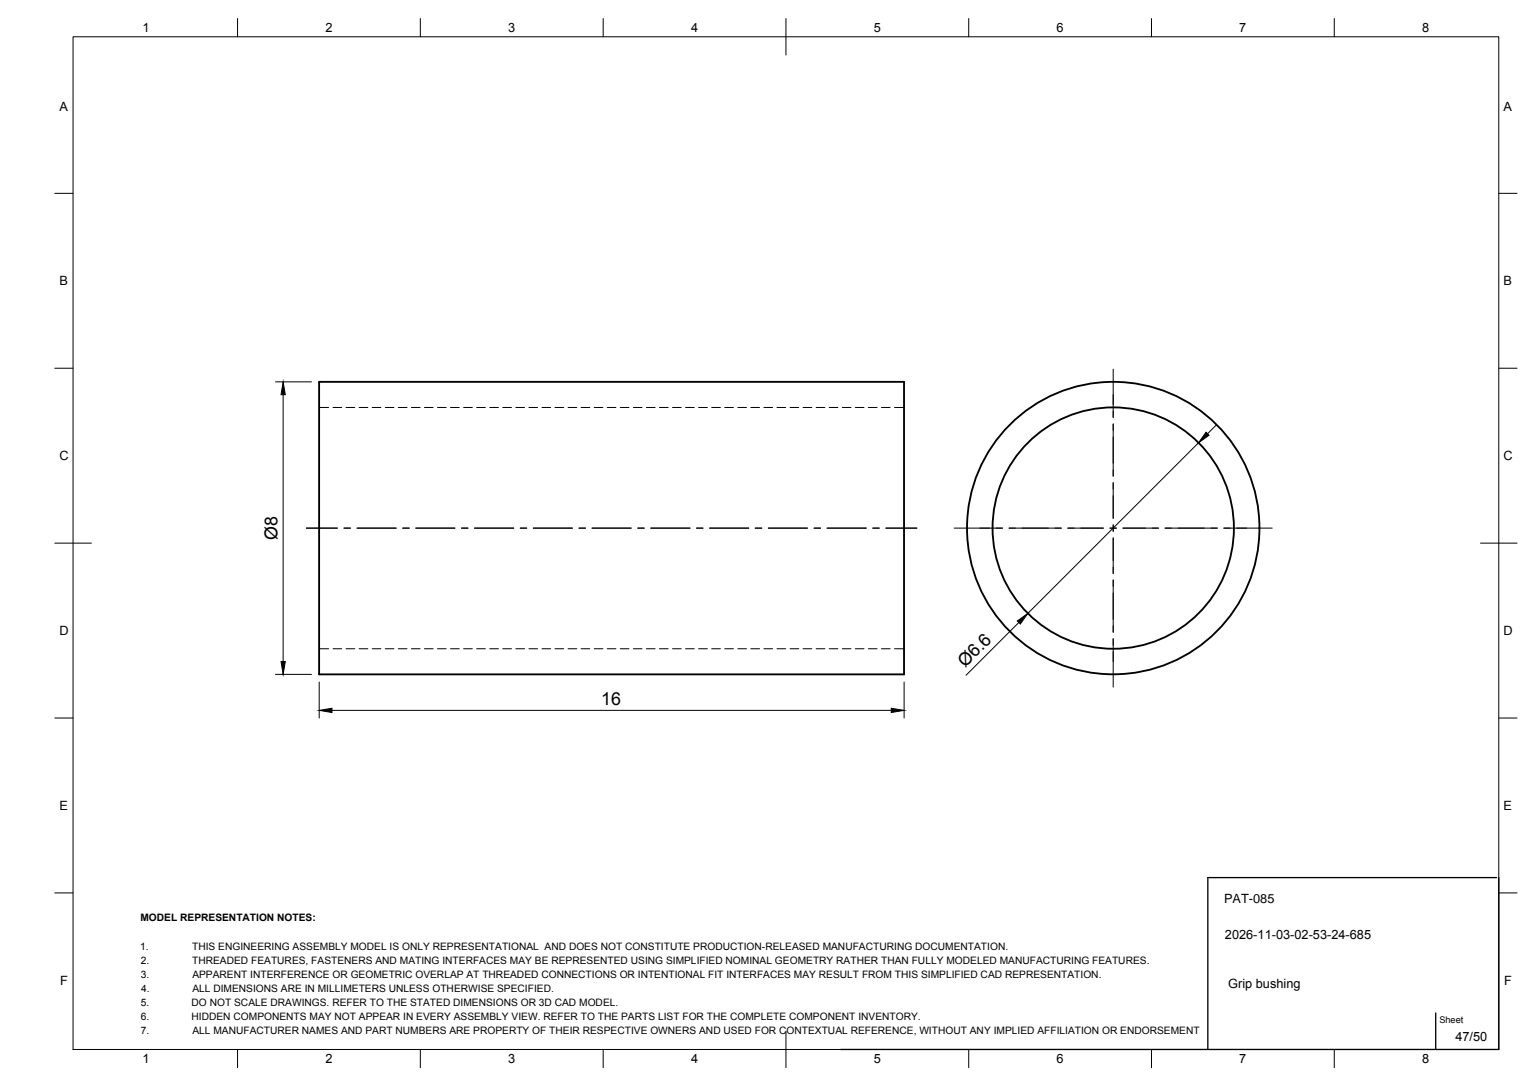
ISO-10303-21;
HEADER;
/* Generated by software containing ST-Developer
 * from STEP Tools, Inc. (www.steptools.com) 
 */

FILE_DESCRIPTION(
/* description */ ('Rack and pinion manual slide'),
/* implementation_level */ '2;1');

FILE_NAME(
/* name */ 'Grip bushing.step',
/* time_stamp */ '2026-10-28T03:22:49-07:00',
/* author */ (''),
/* organization */ (''),
/* preprocessor_version */ 'ST-DEVELOPER v20.2',
/* originating_system */ 'Autodesk Translation Framework v15.17.0.0',
/* authorisation */ '');

FILE_SCHEMA (('AUTOMOTIVE_DESIGN { 1 0 10303 214 3 1 1 }'));
ENDSEC;

DATA;
#10=MECHANICAL_DESIGN_GEOMETRIC_PRESENTATION_REPRESENTATION('',(#778),#34851);
#679=SHAPE_REPRESENTATION_RELATIONSHIP('SRR','None',#35118,#725);
#725=ADVANCED_BREP_SHAPE_REPRESENTATION('',(#828),#34843);
#778=STYLED_ITEM('',(#35418),#828);
#828=MANIFOLD_SOLID_BREP('Body1',#13801);
#1033=FACE_BOUND('',#3072,.T.);
#1034=FACE_BOUND('',#3074,.T.);
#1471=PLANE('',#15320);
#1472=PLANE('',#15321);
#2130=FACE_OUTER_BOUND('',#3069,.T.);
#2131=FACE_OUTER_BOUND('',#3070,.T.);
#2132=FACE_OUTER_BOUND('',#3071,.T.);
#2133=FACE_OUTER_BOUND('',#3073,.T.);
#3069=EDGE_LOOP('',(#12122,#12123,#12124,#12125));
#3070=EDGE_LOOP('',(#12126,#12127,#12128,#12129));
#3071=EDGE_LOOP('',(#12130));
#3072=EDGE_LOOP('',(#12131));
#3073=EDGE_LOOP('',(#12132));
#3074=EDGE_LOOP('',(#12133));
#4306=LINE('',#22815,#5597);
#4307=LINE('',#22821,#5598);
#5597=VECTOR('',#18680,0.33);
#5598=VECTOR('',#18687,0.4);
#6152=CIRCLE('',#15315,0.33);
#6153=CIRCLE('',#15316,0.33);
#6154=CIRCLE('',#15318,0.4);
#6155=CIRCLE('',#15319,0.4);
#7191=VERTEX_POINT('',#22812);
#7192=VERTEX_POINT('',#22814);
#7193=VERTEX_POINT('',#22818);
#7194=VERTEX_POINT('',#22820);
#8873=EDGE_CURVE('',#7191,#7191,#6152,.T.);
#8874=EDGE_CURVE('',#7191,#7192,#4306,.T.);
#8875=EDGE_CURVE('',#7192,#7192,#6153,.T.);
#8876=EDGE_CURVE('',#7193,#7193,#6154,.T.);
#8877=EDGE_CURVE('',#7193,#7194,#4307,.T.);
#8878=EDGE_CURVE('',#7194,#7194,#6155,.T.);
#12122=ORIENTED_EDGE('',*,*,#8873,.F.);
#12123=ORIENTED_EDGE('',*,*,#8874,.T.);
#12124=ORIENTED_EDGE('',*,*,#8875,.T.);
#12125=ORIENTED_EDGE('',*,*,#8874,.F.);
#12126=ORIENTED_EDGE('',*,*,#8876,.F.);
#12127=ORIENTED_EDGE('',*,*,#8877,.T.);
#12128=ORIENTED_EDGE('',*,*,#8878,.T.);
#12129=ORIENTED_EDGE('',*,*,#8877,.F.);
#12130=ORIENTED_EDGE('',*,*,#8876,.T.);
#12131=ORIENTED_EDGE('',*,*,#8873,.T.);
#12132=ORIENTED_EDGE('',*,*,#8878,.F.);
#12133=ORIENTED_EDGE('',*,*,#8875,.F.);
#12981=CYLINDRICAL_SURFACE('',#15314,0.33);
#12982=CYLINDRICAL_SURFACE('',#15317,0.4);
#13608=ADVANCED_FACE('',(#2130),#12981,.F.);
#13609=ADVANCED_FACE('',(#2131),#12982,.T.);
#13610=ADVANCED_FACE('',(#2132,#1033),#1471,.T.);
#13611=ADVANCED_FACE('',(#2133,#1034),#1472,.F.);
#13801=CLOSED_SHELL('',(#13608,#13609,#13610,#13611));
#15313=AXIS2_PLACEMENT_3D('',#22810,#18674,#18675);
#15314=AXIS2_PLACEMENT_3D('',#22811,#18676,#18677);
#15315=AXIS2_PLACEMENT_3D('',#22813,#18678,#18679);
#15316=AXIS2_PLACEMENT_3D('',#22816,#18681,#18682);
#15317=AXIS2_PLACEMENT_3D('',#22817,#18683,#18684);
#15318=AXIS2_PLACEMENT_3D('',#22819,#18685,#18686);
#15319=AXIS2_PLACEMENT_3D('',#22822,#18688,#18689);
#15320=AXIS2_PLACEMENT_3D('',#22823,#18690,#18691);
#15321=AXIS2_PLACEMENT_3D('',#22824,#18692,#18693);
#18674=DIRECTION('axis',(0.,0.,1.));
#18675=DIRECTION('refdir',(1.,0.,0.));
#18676=DIRECTION('center_axis',(0.,1.,0.));
#18677=DIRECTION('ref_axis',(1.,0.,0.));
#18678=DIRECTION('center_axis',(0.,-1.,0.));
#18679=DIRECTION('ref_axis',(1.,0.,0.));
#18680=DIRECTION('',(0.,-1.,0.));
#18681=DIRECTION('center_axis',(0.,-1.,0.));
#18682=DIRECTION('ref_axis',(1.,0.,0.));
#18683=DIRECTION('center_axis',(0.,1.,0.));
#18684=DIRECTION('ref_axis',(1.,0.,0.));
#18685=DIRECTION('center_axis',(0.,1.,0.));
#18686=DIRECTION('ref_axis',(1.,0.,0.));
#18687=DIRECTION('',(0.,-1.,0.));
#18688=DIRECTION('center_axis',(0.,1.,0.));
#18689=DIRECTION('ref_axis',(1.,0.,0.));
#18690=DIRECTION('center_axis',(0.,1.,0.));
#18691=DIRECTION('ref_axis',(1.,0.,0.));
#18692=DIRECTION('center_axis',(0.,1.,0.));
#18693=DIRECTION('ref_axis',(1.,0.,0.));
#22810=CARTESIAN_POINT('',(0.,0.,0.));
#22811=CARTESIAN_POINT('Origin',(11.,7.3,13.25));
#22812=CARTESIAN_POINT('',(10.67,8.9,13.25));
#22813=CARTESIAN_POINT('Origin',(11.,8.9,13.25));
#22814=CARTESIAN_POINT('',(10.67,7.3,13.25));
#22815=CARTESIAN_POINT('',(10.67,7.3,13.25));
#22816=CARTESIAN_POINT('Origin',(11.,7.3,13.25));
#22817=CARTESIAN_POINT('Origin',(11.,7.3,13.25));
#22818=CARTESIAN_POINT('',(10.6,8.9,13.25));
#22819=CARTESIAN_POINT('Origin',(11.,8.9,13.25));
#22820=CARTESIAN_POINT('',(10.6,7.3,13.25));
#22821=CARTESIAN_POINT('',(10.6,7.3,13.25));
#22822=CARTESIAN_POINT('Origin',(11.,7.3,13.25));
#22823=CARTESIAN_POINT('Origin',(11.,8.9,13.25));
#22824=CARTESIAN_POINT('Origin',(11.,7.3,13.25));
#34789=UNCERTAINTY_MEASURE_WITH_UNIT(LENGTH_MEASURE(0.001),#34852,
'DISTANCE_ACCURACY_VALUE',
'Maximum model space distance between geometric entities at asserted c
onnectivities');
#34797=UNCERTAINTY_MEASURE_WITH_UNIT(LENGTH_MEASURE(0.001),#34852,
'DISTANCE_ACCURACY_VALUE',
'Maximum model space distance between geometric entities at asserted c
onnectivities');
#34843=(
GEOMETRIC_REPRESENTATION_CONTEXT(3)
GLOBAL_UNCERTAINTY_ASSIGNED_CONTEXT((#34789))
GLOBAL_UNIT_ASSIGNED_CONTEXT((#34852,#34854,#34855))
REPRESENTATION_CONTEXT('','3D')
);
#34851=(
GEOMETRIC_REPRESENTATION_CONTEXT(3)
GLOBAL_UNCERTAINTY_ASSIGNED_CONTEXT((#34797))
GLOBAL_UNIT_ASSIGNED_CONTEXT((#34852,#34854,#34855))
REPRESENTATION_CONTEXT('','3D')
);
#34852=(
LENGTH_UNIT()
NAMED_UNIT(*)
SI_UNIT(.CENTI.,.METRE.)
);
#34854=(
NAMED_UNIT(*)
PLANE_ANGLE_UNIT()
SI_UNIT($,.RADIAN.)
);
#34855=(
NAMED_UNIT(*)
SI_UNIT($,.STERADIAN.)
SOLID_ANGLE_UNIT()
);
#34901=SHAPE_DEFINITION_REPRESENTATION(#34962,#35118);
#34962=PRODUCT_DEFINITION_SHAPE('',$,#35172);
#35118=SHAPE_REPRESENTATION('',(#15313),#34843);
#35126=PRODUCT_DEFINITION_CONTEXT('part definition',#35287,'design');
#35172=PRODUCT_DEFINITION('Grip bushing','Grip bushing',#35225,#35126);
#35225=PRODUCT_DEFINITION_FORMATION('',$,#35334);
#35287=APPLICATION_CONTEXT(
'Core Data for Automotive Mechanical Design Process');
#35288=PRODUCT_CONTEXT('part definition',#35287,'mechanical');
#35334=PRODUCT('Grip bushing','Grip bushing','Grip bushing',(#35288));
#35412=COLOUR_RGB('Black',0.12,0.14,0.17);
#35413=FILL_AREA_STYLE_COLOUR('',#35412);
#35414=FILL_AREA_STYLE('',(#35413));
#35415=SURFACE_STYLE_FILL_AREA(#35414);
#35416=SURFACE_SIDE_STYLE('',(#35415));
#35417=SURFACE_STYLE_USAGE(.BOTH.,#35416);
#35418=PRESENTATION_STYLE_ASSIGNMENT((#35417));
ENDSEC;
END-ISO-10303-21;
